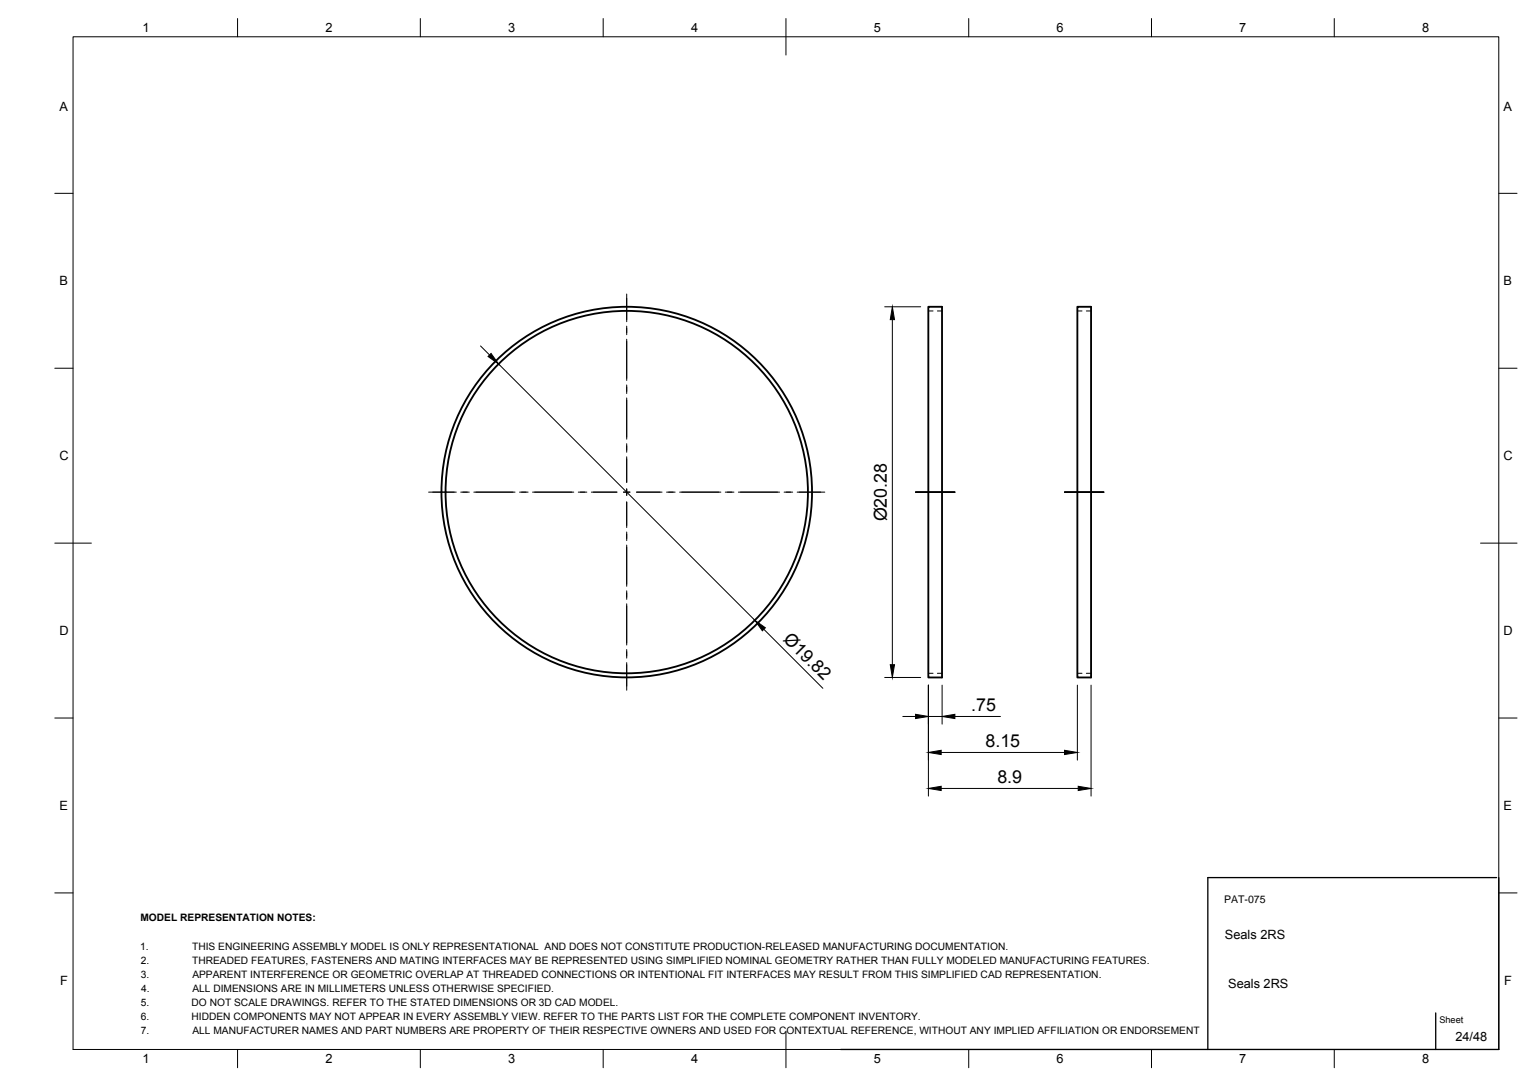
ISO-10303-21;
HEADER;
/* Generated by software containing ST-Developer
 * from STEP Tools, Inc. (www.steptools.com) 
 */

FILE_DESCRIPTION(
/* description */ ('Over-Centre Plunger Toggle Clamp on Slotted Fixture Frame'),
/* implementation_level */ '2;1');

FILE_NAME(
/* name */ 
'Seals 2RS.step',
/* time_stamp */ '2026-10-28T03:23:24-07:00',
/* author */ (''),
/* organization */ (''),
/* preprocessor_version */ 'ST-DEVELOPER v20.2',
/* originating_system */ 'Autodesk Translation Framework v15.17.0.0',
/* authorisation */ '');

FILE_SCHEMA (('AUTOMOTIVE_DESIGN { 1 0 10303 214 3 1 1 }'));
ENDSEC;

DATA;
#10=MECHANICAL_DESIGN_GEOMETRIC_PRESENTATION_REPRESENTATION('',(#540,#541),#15212);
#449=SHAPE_REPRESENTATION_RELATIONSHIP('SRR','None',#15424,#491);
#491=ADVANCED_BREP_SHAPE_REPRESENTATION('',(#590,#591),#15186);
#540=STYLED_ITEM('',(#15719),#590);
#541=STYLED_ITEM('',(#15719),#591);
#590=MANIFOLD_SOLID_BREP('Body1',#8273);
#591=MANIFOLD_SOLID_BREP('Body2',#8274);
#725=FACE_BOUND('',#1962,.T.);
#726=FACE_BOUND('',#1965,.T.);
#727=FACE_BOUND('',#1968,.T.);
#728=FACE_BOUND('',#1971,.T.);
#951=PLANE('',#9277);
#952=PLANE('',#9282);
#953=PLANE('',#9285);
#954=PLANE('',#9290);
#1361=FACE_OUTER_BOUND('',#1961,.T.);
#1362=FACE_OUTER_BOUND('',#1963,.T.);
#1363=FACE_OUTER_BOUND('',#1964,.T.);
#1364=FACE_OUTER_BOUND('',#1966,.T.);
#1365=FACE_OUTER_BOUND('',#1967,.T.);
#1366=FACE_OUTER_BOUND('',#1969,.T.);
#1367=FACE_OUTER_BOUND('',#1970,.T.);
#1368=FACE_OUTER_BOUND('',#1972,.T.);
#1961=EDGE_LOOP('',(#6817));
#1962=EDGE_LOOP('',(#6818));
#1963=EDGE_LOOP('',(#6819,#6820,#6821,#6822));
#1964=EDGE_LOOP('',(#6823));
#1965=EDGE_LOOP('',(#6824));
#1966=EDGE_LOOP('',(#6825,#6826,#6827,#6828));
#1967=EDGE_LOOP('',(#6829));
#1968=EDGE_LOOP('',(#6830));
#1969=EDGE_LOOP('',(#6831,#6832,#6833,#6834));
#1970=EDGE_LOOP('',(#6835));
#1971=EDGE_LOOP('',(#6836));
#1972=EDGE_LOOP('',(#6837,#6838,#6839,#6840));
#2621=LINE('',#14058,#3251);
#2622=LINE('',#14063,#3252);
#2623=LINE('',#14072,#3253);
#2624=LINE('',#14077,#3254);
#3251=VECTOR('',#11182,1.013815);
#3252=VECTOR('',#11189,0.991185);
#3253=VECTOR('',#11200,1.013815);
#3254=VECTOR('',#11207,0.991185);
#3705=CIRCLE('',#9278,1.013815);
#3706=CIRCLE('',#9279,0.991185);
#3707=CIRCLE('',#9281,1.013815);
#3708=CIRCLE('',#9283,0.991185);
#3709=CIRCLE('',#9286,1.013815);
#3710=CIRCLE('',#9287,0.991185);
#3711=CIRCLE('',#9289,1.013815);
#3712=CIRCLE('',#9291,0.991185);
#4283=VERTEX_POINT('',#14051);
#4284=VERTEX_POINT('',#14053);
#4285=VERTEX_POINT('',#14056);
#4286=VERTEX_POINT('',#14060);
#4287=VERTEX_POINT('',#14065);
#4288=VERTEX_POINT('',#14067);
#4289=VERTEX_POINT('',#14070);
#4290=VERTEX_POINT('',#14074);
#5169=EDGE_CURVE('',#4283,#4283,#3705,.T.);
#5170=EDGE_CURVE('',#4284,#4284,#3706,.T.);
#5171=EDGE_CURVE('',#4285,#4285,#3707,.T.);
#5172=EDGE_CURVE('',#4285,#4283,#2621,.T.);
#5173=EDGE_CURVE('',#4286,#4286,#3708,.T.);
#5174=EDGE_CURVE('',#4286,#4284,#2622,.T.);
#5175=EDGE_CURVE('',#4287,#4287,#3709,.T.);
#5176=EDGE_CURVE('',#4288,#4288,#3710,.T.);
#5177=EDGE_CURVE('',#4289,#4289,#3711,.T.);
#5178=EDGE_CURVE('',#4289,#4287,#2623,.T.);
#5179=EDGE_CURVE('',#4290,#4290,#3712,.T.);
#5180=EDGE_CURVE('',#4290,#4288,#2624,.T.);
#6817=ORIENTED_EDGE('',*,*,#5169,.F.);
#6818=ORIENTED_EDGE('',*,*,#5170,.T.);
#6819=ORIENTED_EDGE('',*,*,#5171,.F.);
#6820=ORIENTED_EDGE('',*,*,#5172,.T.);
#6821=ORIENTED_EDGE('',*,*,#5169,.T.);
#6822=ORIENTED_EDGE('',*,*,#5172,.F.);
#6823=ORIENTED_EDGE('',*,*,#5171,.T.);
#6824=ORIENTED_EDGE('',*,*,#5173,.F.);
#6825=ORIENTED_EDGE('',*,*,#5173,.T.);
#6826=ORIENTED_EDGE('',*,*,#5174,.T.);
#6827=ORIENTED_EDGE('',*,*,#5170,.F.);
#6828=ORIENTED_EDGE('',*,*,#5174,.F.);
#6829=ORIENTED_EDGE('',*,*,#5175,.F.);
#6830=ORIENTED_EDGE('',*,*,#5176,.T.);
#6831=ORIENTED_EDGE('',*,*,#5177,.F.);
#6832=ORIENTED_EDGE('',*,*,#5178,.T.);
#6833=ORIENTED_EDGE('',*,*,#5175,.T.);
#6834=ORIENTED_EDGE('',*,*,#5178,.F.);
#6835=ORIENTED_EDGE('',*,*,#5177,.T.);
#6836=ORIENTED_EDGE('',*,*,#5179,.F.);
#6837=ORIENTED_EDGE('',*,*,#5179,.T.);
#6838=ORIENTED_EDGE('',*,*,#5180,.T.);
#6839=ORIENTED_EDGE('',*,*,#5176,.F.);
#6840=ORIENTED_EDGE('',*,*,#5180,.F.);
#7697=CYLINDRICAL_SURFACE('',#9280,1.013815);
#7698=CYLINDRICAL_SURFACE('',#9284,0.991185);
#7699=CYLINDRICAL_SURFACE('',#9288,1.013815);
#7700=CYLINDRICAL_SURFACE('',#9292,0.991185);
#8033=ADVANCED_FACE('',(#1361,#725),#951,.T.);
#8034=ADVANCED_FACE('',(#1362),#7697,.T.);
#8035=ADVANCED_FACE('',(#1363,#726),#952,.T.);
#8036=ADVANCED_FACE('',(#1364),#7698,.F.);
#8037=ADVANCED_FACE('',(#1365,#727),#953,.T.);
#8038=ADVANCED_FACE('',(#1366),#7699,.T.);
#8039=ADVANCED_FACE('',(#1367,#728),#954,.T.);
#8040=ADVANCED_FACE('',(#1368),#7700,.F.);
#8273=CLOSED_SHELL('',(#8033,#8034,#8035,#8036));
#8274=CLOSED_SHELL('',(#8037,#8038,#8039,#8040));
#9276=AXIS2_PLACEMENT_3D('',#14049,#11170,#11171);
#9277=AXIS2_PLACEMENT_3D('',#14050,#11172,#11173);
#9278=AXIS2_PLACEMENT_3D('',#14052,#11174,#11175);
#9279=AXIS2_PLACEMENT_3D('',#14054,#11176,#11177);
#9280=AXIS2_PLACEMENT_3D('',#14055,#11178,#11179);
#9281=AXIS2_PLACEMENT_3D('',#14057,#11180,#11181);
#9282=AXIS2_PLACEMENT_3D('',#14059,#11183,#11184);
#9283=AXIS2_PLACEMENT_3D('',#14061,#11185,#11186);
#9284=AXIS2_PLACEMENT_3D('',#14062,#11187,#11188);
#9285=AXIS2_PLACEMENT_3D('',#14064,#11190,#11191);
#9286=AXIS2_PLACEMENT_3D('',#14066,#11192,#11193);
#9287=AXIS2_PLACEMENT_3D('',#14068,#11194,#11195);
#9288=AXIS2_PLACEMENT_3D('',#14069,#11196,#11197);
#9289=AXIS2_PLACEMENT_3D('',#14071,#11198,#11199);
#9290=AXIS2_PLACEMENT_3D('',#14073,#11201,#11202);
#9291=AXIS2_PLACEMENT_3D('',#14075,#11203,#11204);
#9292=AXIS2_PLACEMENT_3D('',#14076,#11205,#11206);
#11170=DIRECTION('axis',(0.,0.,1.));
#11171=DIRECTION('refdir',(1.,0.,0.));
#11172=DIRECTION('center_axis',(0.,1.,0.));
#11173=DIRECTION('ref_axis',(0.,0.,1.));
#11174=DIRECTION('center_axis',(0.,-1.,0.));
#11175=DIRECTION('ref_axis',(1.,0.,0.));
#11176=DIRECTION('center_axis',(0.,-1.,0.));
#11177=DIRECTION('ref_axis',(1.,0.,0.));
#11178=DIRECTION('center_axis',(0.,-1.,0.));
#11179=DIRECTION('ref_axis',(1.,0.,0.));
#11180=DIRECTION('center_axis',(0.,-1.,0.));
#11181=DIRECTION('ref_axis',(1.,0.,0.));
#11182=DIRECTION('',(0.,1.,0.));
#11183=DIRECTION('center_axis',(0.,-1.,0.));
#11184=DIRECTION('ref_axis',(0.,0.,-1.));
#11185=DIRECTION('center_axis',(0.,-1.,0.));
#11186=DIRECTION('ref_axis',(1.,0.,0.));
#11187=DIRECTION('center_axis',(0.,-1.,0.));
#11188=DIRECTION('ref_axis',(1.,0.,0.));
#11189=DIRECTION('',(0.,1.,0.));
#11190=DIRECTION('center_axis',(0.,1.,0.));
#11191=DIRECTION('ref_axis',(0.,0.,1.));
#11192=DIRECTION('center_axis',(0.,-1.,0.));
#11193=DIRECTION('ref_axis',(1.,0.,0.));
#11194=DIRECTION('center_axis',(0.,-1.,0.));
#11195=DIRECTION('ref_axis',(1.,0.,0.));
#11196=DIRECTION('center_axis',(0.,-1.,0.));
#11197=DIRECTION('ref_axis',(1.,0.,0.));
#11198=DIRECTION('center_axis',(0.,-1.,0.));
#11199=DIRECTION('ref_axis',(1.,0.,0.));
#11200=DIRECTION('',(0.,1.,0.));
#11201=DIRECTION('center_axis',(0.,-1.,0.));
#11202=DIRECTION('ref_axis',(0.,0.,-1.));
#11203=DIRECTION('center_axis',(0.,-1.,0.));
#11204=DIRECTION('ref_axis',(1.,0.,0.));
#11205=DIRECTION('center_axis',(0.,-1.,0.));
#11206=DIRECTION('ref_axis',(1.,0.,0.));
#11207=DIRECTION('',(0.,1.,0.));
#14049=CARTESIAN_POINT('',(0.,0.,0.));
#14050=CARTESIAN_POINT('Origin',(1.013815,0.445,0.));
#14051=CARTESIAN_POINT('',(-1.013815,0.445,-1.24156529467757E-16));
#14052=CARTESIAN_POINT('Origin',(0.,0.445,0.));
#14053=CARTESIAN_POINT('',(-0.991185,0.445,-1.21385153761287E-16));
#14054=CARTESIAN_POINT('Origin',(0.,0.445,0.));
#14055=CARTESIAN_POINT('Origin',(0.,0.4075,0.));
#14056=CARTESIAN_POINT('',(-1.013815,0.37,-1.24156529467757E-16));
#14057=CARTESIAN_POINT('Origin',(0.,0.37,0.));
#14058=CARTESIAN_POINT('',(-1.013815,0.4075,-1.24156529467757E-16));
#14059=CARTESIAN_POINT('Origin',(0.991185,0.37,0.));
#14060=CARTESIAN_POINT('',(-0.991185,0.37,-1.21385153761287E-16));
#14061=CARTESIAN_POINT('Origin',(0.,0.37,0.));
#14062=CARTESIAN_POINT('Origin',(0.,0.4075,0.));
#14063=CARTESIAN_POINT('',(-0.991185,0.4075,-1.21385153761287E-16));
#14064=CARTESIAN_POINT('Origin',(1.013815,-0.37,0.));
#14065=CARTESIAN_POINT('',(-1.013815,-0.37,-1.24156529467757E-16));
#14066=CARTESIAN_POINT('Origin',(0.,-0.37,0.));
#14067=CARTESIAN_POINT('',(-0.991185,-0.37,-1.21385153761287E-16));
#14068=CARTESIAN_POINT('Origin',(0.,-0.37,0.));
#14069=CARTESIAN_POINT('Origin',(0.,-0.4075,0.));
#14070=CARTESIAN_POINT('',(-1.013815,-0.445,-1.24156529467757E-16));
#14071=CARTESIAN_POINT('Origin',(0.,-0.445,0.));
#14072=CARTESIAN_POINT('',(-1.013815,-0.4075,-1.24156529467757E-16));
#14073=CARTESIAN_POINT('Origin',(0.991185,-0.445,0.));
#14074=CARTESIAN_POINT('',(-0.991185,-0.445,-1.21385153761287E-16));
#14075=CARTESIAN_POINT('Origin',(0.,-0.445,0.));
#14076=CARTESIAN_POINT('Origin',(0.,-0.4075,0.));
#14077=CARTESIAN_POINT('',(-0.991185,-0.4075,-1.21385153761287E-16));
#15136=UNCERTAINTY_MEASURE_WITH_UNIT(LENGTH_MEASURE(0.001),#15213,
'DISTANCE_ACCURACY_VALUE',
'Maximum model space distance between geometric entities at asserted c
onnectivities');
#15162=UNCERTAINTY_MEASURE_WITH_UNIT(LENGTH_MEASURE(0.001),#15213,
'DISTANCE_ACCURACY_VALUE',
'Maximum model space distance between geometric entities at asserted c
onnectivities');
#15186=(
GEOMETRIC_REPRESENTATION_CONTEXT(3)
GLOBAL_UNCERTAINTY_ASSIGNED_CONTEXT((#15136))
GLOBAL_UNIT_ASSIGNED_CONTEXT((#15213,#15215,#15216))
REPRESENTATION_CONTEXT('','3D')
);
#15212=(
GEOMETRIC_REPRESENTATION_CONTEXT(3)
GLOBAL_UNCERTAINTY_ASSIGNED_CONTEXT((#15162))
GLOBAL_UNIT_ASSIGNED_CONTEXT((#15213,#15215,#15216))
REPRESENTATION_CONTEXT('','3D')
);
#15213=(
LENGTH_UNIT()
NAMED_UNIT(*)
SI_UNIT(.CENTI.,.METRE.)
);
#15215=(
NAMED_UNIT(*)
PLANE_ANGLE_UNIT()
SI_UNIT($,.RADIAN.)
);
#15216=(
NAMED_UNIT(*)
SI_UNIT($,.STERADIAN.)
SOLID_ANGLE_UNIT()
);
#15240=SHAPE_DEFINITION_REPRESENTATION(#15289,#15424);
#15289=PRODUCT_DEFINITION_SHAPE('',$,#15474);
#15424=SHAPE_REPRESENTATION('',(#9276),#15186);
#15450=PRODUCT_DEFINITION_CONTEXT('part definition',#15599,'design');
#15474=PRODUCT_DEFINITION('Seals 2RS','Seals 2RS',#15523,#15450);
#15523=PRODUCT_DEFINITION_FORMATION('',$,#15624);
#15599=APPLICATION_CONTEXT(
'Core Data for Automotive Mechanical Design Process');
#15600=PRODUCT_CONTEXT('part definition',#15599,'mechanical');
#15624=PRODUCT('Seals 2RS','Seals 2RS','Seals 2RS',(#15600));
#15713=COLOUR_RGB('Grey',0.48,0.52,0.57);
#15714=FILL_AREA_STYLE_COLOUR('',#15713);
#15715=FILL_AREA_STYLE('',(#15714));
#15716=SURFACE_STYLE_FILL_AREA(#15715);
#15717=SURFACE_SIDE_STYLE('',(#15716));
#15718=SURFACE_STYLE_USAGE(.BOTH.,#15717);
#15719=PRESENTATION_STYLE_ASSIGNMENT((#15718));
ENDSEC;
END-ISO-10303-21;
